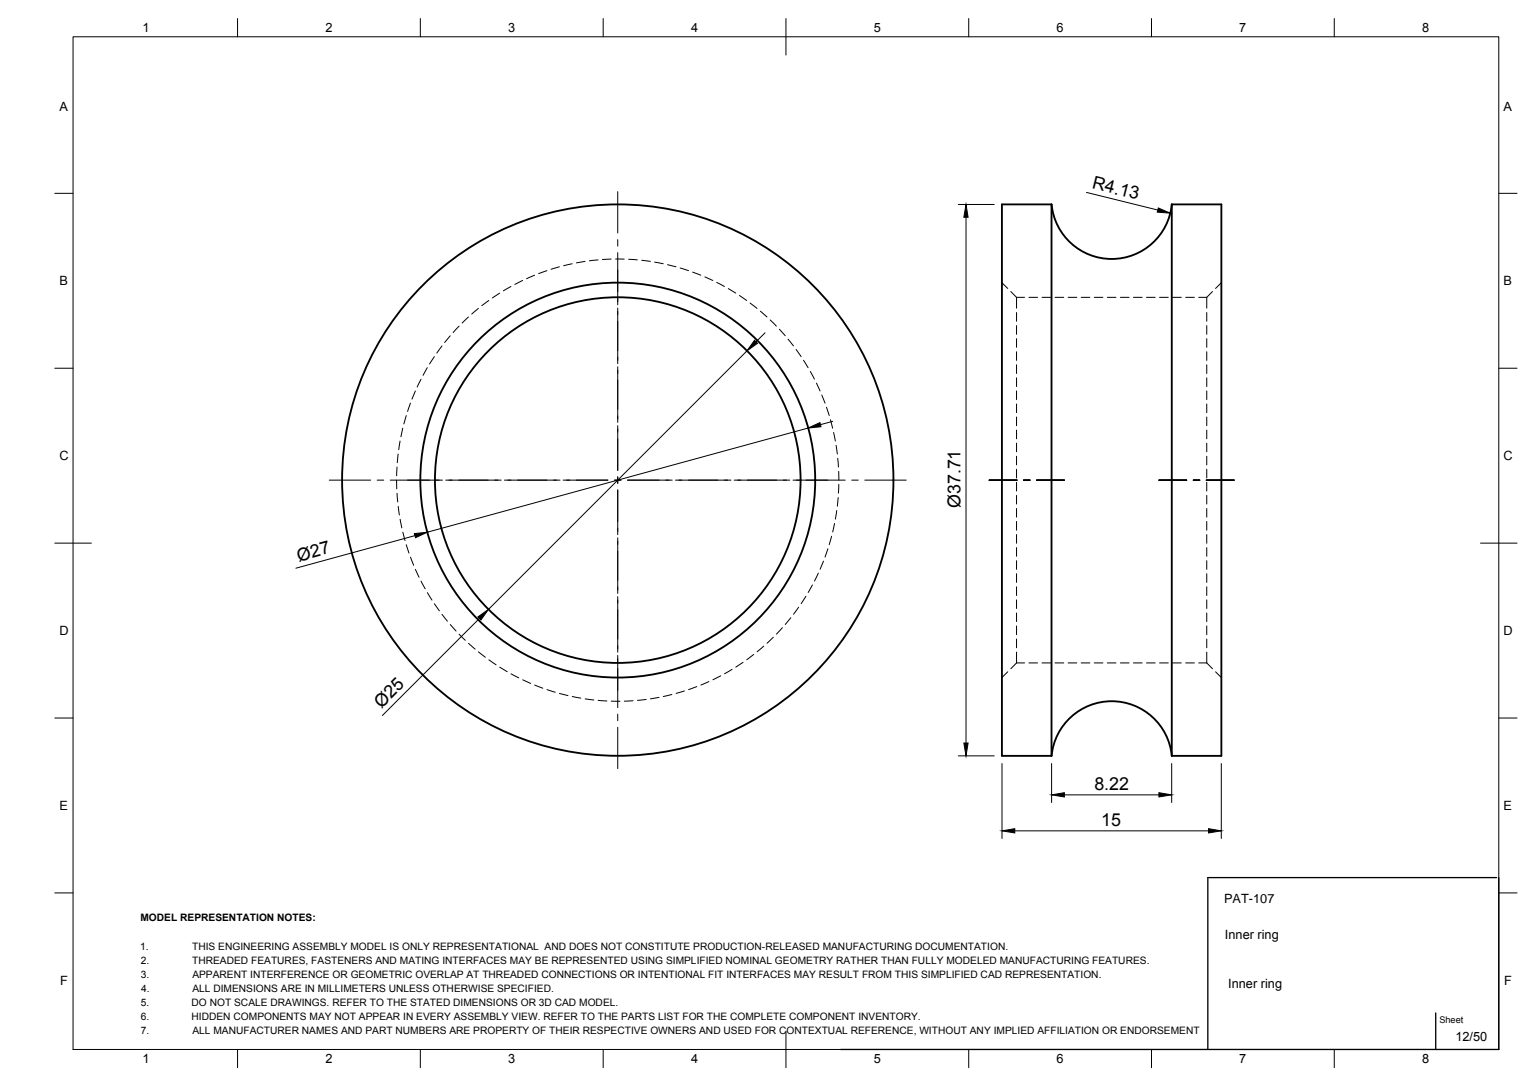
ISO-10303-21;
HEADER;
/* Generated by software containing ST-Developer
 * from STEP Tools, Inc. (www.steptools.com) 
 */

FILE_DESCRIPTION(
/* description */ ('Turntable on roller ring'),
/* implementation_level */ '2;1');

FILE_NAME(
/* name */ 'Inner ring.step',
/* time_stamp */ '2026-10-28T03:23:59-07:00',
/* author */ (''),
/* organization */ (''),
/* preprocessor_version */ 'ST-DEVELOPER v20.2',
/* originating_system */ 'Autodesk Translation Framework v15.17.0.0',
/* authorisation */ '');

FILE_SCHEMA (('AUTOMOTIVE_DESIGN { 1 0 10303 214 3 1 1 }'));
ENDSEC;

DATA;
#10=MECHANICAL_DESIGN_GEOMETRIC_PRESENTATION_REPRESENTATION('',(#621),#16281);
#472=TOROIDAL_SURFACE('',#9232,1.925,0.412776);
#479=CONICAL_SURFACE('',#9243,1.3,0.785398163397449);
#480=CONICAL_SURFACE('',#9250,1.3,0.785398163397449);
#511=SHAPE_REPRESENTATION_RELATIONSHIP('SRR','None',#16526,#566);
#566=ADVANCED_BREP_SHAPE_REPRESENTATION('',(#692),#16220);
#621=STYLED_ITEM('',(#16932),#692);
#692=MANIFOLD_SOLID_BREP('Body1',#8363);
#824=FACE_BOUND('',#1909,.T.);
#825=FACE_BOUND('',#1912,.T.);
#1021=PLANE('',#9245);
#1022=PLANE('',#9248);
#1332=FACE_OUTER_BOUND('',#1904,.T.);
#1333=FACE_OUTER_BOUND('',#1905,.T.);
#1334=FACE_OUTER_BOUND('',#1906,.T.);
#1335=FACE_OUTER_BOUND('',#1907,.T.);
#1336=FACE_OUTER_BOUND('',#1908,.T.);
#1337=FACE_OUTER_BOUND('',#1910,.T.);
#1338=FACE_OUTER_BOUND('',#1911,.T.);
#1339=FACE_OUTER_BOUND('',#1913,.T.);
#1904=EDGE_LOOP('',(#6019,#6020,#6021,#6022,#6023,#6024));
#1905=EDGE_LOOP('',(#6025,#6026,#6027,#6028,#6029));
#1906=EDGE_LOOP('',(#6030,#6031,#6032,#6033));
#1907=EDGE_LOOP('',(#6034,#6035,#6036,#6037));
#1908=EDGE_LOOP('',(#6038));
#1909=EDGE_LOOP('',(#6039));
#1910=EDGE_LOOP('',(#6040,#6041,#6042,#6043,#6044));
#1911=EDGE_LOOP('',(#6045));
#1912=EDGE_LOOP('',(#6046));
#1913=EDGE_LOOP('',(#6047,#6048,#6049,#6050));
#2578=LINE('',#13410,#3061);
#2579=LINE('',#13416,#3062);
#2580=LINE('',#13420,#3063);
#2581=LINE('',#13426,#3064);
#2582=LINE('',#13431,#3065);
#3061=VECTOR('',#10683,1.88531);
#3062=VECTOR('',#10690,1.25);
#3063=VECTOR('',#10695,1.3);
#3064=VECTOR('',#10704,1.88531);
#3065=VECTOR('',#10711,1.3);
#3561=CIRCLE('',#9233,1.88531);
#3562=CIRCLE('',#9234,1.88531);
#3563=CIRCLE('',#9235,0.412776);
#3564=CIRCLE('',#9236,1.88531);
#3565=CIRCLE('',#9237,1.88531);
#3566=CIRCLE('',#9239,1.88531);
#3567=CIRCLE('',#9241,1.25);
#3568=CIRCLE('',#9242,1.25);
#3569=CIRCLE('',#9244,1.35);
#3570=CIRCLE('',#9247,1.88531);
#3571=CIRCLE('',#9249,1.35);
#4067=VERTEX_POINT('',#13399);
#4068=VERTEX_POINT('',#13400);
#4069=VERTEX_POINT('',#13403);
#4070=VERTEX_POINT('',#13405);
#4071=VERTEX_POINT('',#13409);
#4072=VERTEX_POINT('',#13413);
#4073=VERTEX_POINT('',#13415);
#4074=VERTEX_POINT('',#13419);
#4075=VERTEX_POINT('',#13424);
#4076=VERTEX_POINT('',#13428);
#4820=EDGE_CURVE('',#4067,#4068,#3561,.T.);
#4821=EDGE_CURVE('',#4068,#4067,#3562,.T.);
#4822=EDGE_CURVE('',#4068,#4069,#3563,.T.);
#4823=EDGE_CURVE('',#4070,#4069,#3564,.T.);
#4824=EDGE_CURVE('',#4069,#4070,#3565,.T.);
#4825=EDGE_CURVE('',#4070,#4071,#2578,.T.);
#4826=EDGE_CURVE('',#4071,#4071,#3566,.T.);
#4827=EDGE_CURVE('',#4072,#4072,#3567,.T.);
#4828=EDGE_CURVE('',#4072,#4073,#2579,.T.);
#4829=EDGE_CURVE('',#4073,#4073,#3568,.T.);
#4830=EDGE_CURVE('',#4073,#4074,#2580,.T.);
#4831=EDGE_CURVE('',#4074,#4074,#3569,.T.);
#4832=EDGE_CURVE('',#4075,#4075,#3570,.T.);
#4833=EDGE_CURVE('',#4075,#4067,#2581,.T.);
#4834=EDGE_CURVE('',#4076,#4076,#3571,.T.);
#4835=EDGE_CURVE('',#4076,#4072,#2582,.T.);
#6019=ORIENTED_EDGE('',*,*,#4820,.F.);
#6020=ORIENTED_EDGE('',*,*,#4821,.F.);
#6021=ORIENTED_EDGE('',*,*,#4822,.T.);
#6022=ORIENTED_EDGE('',*,*,#4823,.F.);
#6023=ORIENTED_EDGE('',*,*,#4824,.F.);
#6024=ORIENTED_EDGE('',*,*,#4822,.F.);
#6025=ORIENTED_EDGE('',*,*,#4823,.T.);
#6026=ORIENTED_EDGE('',*,*,#4824,.T.);
#6027=ORIENTED_EDGE('',*,*,#4825,.T.);
#6028=ORIENTED_EDGE('',*,*,#4826,.T.);
#6029=ORIENTED_EDGE('',*,*,#4825,.F.);
#6030=ORIENTED_EDGE('',*,*,#4827,.T.);
#6031=ORIENTED_EDGE('',*,*,#4828,.T.);
#6032=ORIENTED_EDGE('',*,*,#4829,.F.);
#6033=ORIENTED_EDGE('',*,*,#4828,.F.);
#6034=ORIENTED_EDGE('',*,*,#4829,.T.);
#6035=ORIENTED_EDGE('',*,*,#4830,.T.);
#6036=ORIENTED_EDGE('',*,*,#4831,.F.);
#6037=ORIENTED_EDGE('',*,*,#4830,.F.);
#6038=ORIENTED_EDGE('',*,*,#4826,.F.);
#6039=ORIENTED_EDGE('',*,*,#4831,.T.);
#6040=ORIENTED_EDGE('',*,*,#4832,.F.);
#6041=ORIENTED_EDGE('',*,*,#4833,.T.);
#6042=ORIENTED_EDGE('',*,*,#4820,.T.);
#6043=ORIENTED_EDGE('',*,*,#4821,.T.);
#6044=ORIENTED_EDGE('',*,*,#4833,.F.);
#6045=ORIENTED_EDGE('',*,*,#4832,.T.);
#6046=ORIENTED_EDGE('',*,*,#4834,.F.);
#6047=ORIENTED_EDGE('',*,*,#4834,.T.);
#6048=ORIENTED_EDGE('',*,*,#4835,.T.);
#6049=ORIENTED_EDGE('',*,*,#4827,.F.);
#6050=ORIENTED_EDGE('',*,*,#4835,.F.);
#7717=CYLINDRICAL_SURFACE('',#9238,1.88531);
#7718=CYLINDRICAL_SURFACE('',#9240,1.25);
#7719=CYLINDRICAL_SURFACE('',#9246,1.88531);
#7935=ADVANCED_FACE('',(#1332),#472,.F.);
#7936=ADVANCED_FACE('',(#1333),#7717,.T.);
#7937=ADVANCED_FACE('',(#1334),#7718,.F.);
#7938=ADVANCED_FACE('',(#1335),#479,.F.);
#7939=ADVANCED_FACE('',(#1336,#824),#1021,.T.);
#7940=ADVANCED_FACE('',(#1337),#7719,.T.);
#7941=ADVANCED_FACE('',(#1338,#825),#1022,.T.);
#7942=ADVANCED_FACE('',(#1339),#480,.F.);
#8363=CLOSED_SHELL('',(#7935,#7936,#7937,#7938,#7939,#7940,#7941,#7942));
#9231=AXIS2_PLACEMENT_3D('',#13397,#10667,#10668);
#9232=AXIS2_PLACEMENT_3D('',#13398,#10669,#10670);
#9233=AXIS2_PLACEMENT_3D('',#13401,#10671,#10672);
#9234=AXIS2_PLACEMENT_3D('',#13402,#10673,#10674);
#9235=AXIS2_PLACEMENT_3D('',#13404,#10675,#10676);
#9236=AXIS2_PLACEMENT_3D('',#13406,#10677,#10678);
#9237=AXIS2_PLACEMENT_3D('',#13407,#10679,#10680);
#9238=AXIS2_PLACEMENT_3D('',#13408,#10681,#10682);
#9239=AXIS2_PLACEMENT_3D('',#13411,#10684,#10685);
#9240=AXIS2_PLACEMENT_3D('',#13412,#10686,#10687);
#9241=AXIS2_PLACEMENT_3D('',#13414,#10688,#10689);
#9242=AXIS2_PLACEMENT_3D('',#13417,#10691,#10692);
#9243=AXIS2_PLACEMENT_3D('',#13418,#10693,#10694);
#9244=AXIS2_PLACEMENT_3D('',#13421,#10696,#10697);
#9245=AXIS2_PLACEMENT_3D('',#13422,#10698,#10699);
#9246=AXIS2_PLACEMENT_3D('',#13423,#10700,#10701);
#9247=AXIS2_PLACEMENT_3D('',#13425,#10702,#10703);
#9248=AXIS2_PLACEMENT_3D('',#13427,#10705,#10706);
#9249=AXIS2_PLACEMENT_3D('',#13429,#10707,#10708);
#9250=AXIS2_PLACEMENT_3D('',#13430,#10709,#10710);
#10667=DIRECTION('axis',(0.,0.,1.));
#10668=DIRECTION('refdir',(1.,0.,0.));
#10669=DIRECTION('center_axis',(0.,-1.,0.));
#10670=DIRECTION('ref_axis',(0.,0.,-1.));
#10671=DIRECTION('center_axis',(0.,-1.,0.));
#10672=DIRECTION('ref_axis',(1.,0.,0.));
#10673=DIRECTION('center_axis',(0.,-1.,0.));
#10674=DIRECTION('ref_axis',(1.,0.,0.));
#10675=DIRECTION('center_axis',(1.,0.,1.22464679914735E-16));
#10676=DIRECTION('ref_axis',(-1.22464679914735E-16,0.,1.));
#10677=DIRECTION('center_axis',(0.,1.,0.));
#10678=DIRECTION('ref_axis',(1.,0.,0.));
#10679=DIRECTION('center_axis',(0.,1.,0.));
#10680=DIRECTION('ref_axis',(1.,0.,0.));
#10681=DIRECTION('center_axis',(0.,-1.,0.));
#10682=DIRECTION('ref_axis',(1.,0.,0.));
#10683=DIRECTION('',(0.,1.,0.));
#10684=DIRECTION('center_axis',(0.,-1.,0.));
#10685=DIRECTION('ref_axis',(1.,0.,0.));
#10686=DIRECTION('center_axis',(0.,-1.,0.));
#10687=DIRECTION('ref_axis',(1.,0.,0.));
#10688=DIRECTION('center_axis',(0.,-1.,0.));
#10689=DIRECTION('ref_axis',(1.,0.,0.));
#10690=DIRECTION('',(0.,1.,0.));
#10691=DIRECTION('center_axis',(0.,-1.,0.));
#10692=DIRECTION('ref_axis',(1.,0.,0.));
#10693=DIRECTION('center_axis',(0.,1.,0.));
#10694=DIRECTION('ref_axis',(1.,0.,0.));
#10695=DIRECTION('',(-0.707106781186548,0.707106781186547,-8.65956056235494E-17));
#10696=DIRECTION('center_axis',(0.,-1.,0.));
#10697=DIRECTION('ref_axis',(1.,0.,0.));
#10698=DIRECTION('center_axis',(0.,1.,0.));
#10699=DIRECTION('ref_axis',(0.,0.,1.));
#10700=DIRECTION('center_axis',(0.,-1.,0.));
#10701=DIRECTION('ref_axis',(1.,0.,0.));
#10702=DIRECTION('center_axis',(0.,-1.,0.));
#10703=DIRECTION('ref_axis',(1.,0.,0.));
#10704=DIRECTION('',(0.,1.,0.));
#10705=DIRECTION('center_axis',(0.,-1.,0.));
#10706=DIRECTION('ref_axis',(0.,0.,-1.));
#10707=DIRECTION('center_axis',(0.,-1.,0.));
#10708=DIRECTION('ref_axis',(1.,0.,0.));
#10709=DIRECTION('center_axis',(0.,-1.,0.));
#10710=DIRECTION('ref_axis',(1.,0.,0.));
#10711=DIRECTION('',(0.707106781186548,0.707106781186547,8.65956056235494E-17));
#13397=CARTESIAN_POINT('',(0.,0.,0.));
#13398=CARTESIAN_POINT('Origin',(0.,0.,0.));
#13399=CARTESIAN_POINT('',(-1.88531,-0.410863395882378,-2.3088388569005E-16));
#13400=CARTESIAN_POINT('',(-2.3088388569005E-16,-0.410863395882378,1.88531));
#13401=CARTESIAN_POINT('Origin',(0.,-0.410863395882378,0.));
#13402=CARTESIAN_POINT('Origin',(0.,-0.410863395882378,0.));
#13403=CARTESIAN_POINT('',(-2.3088388569005E-16,0.410863395882378,1.88531));
#13404=CARTESIAN_POINT('Origin',(-2.35744508835865E-16,0.,1.925));
#13405=CARTESIAN_POINT('',(-1.88531,0.410863395882378,2.3088388569005E-16));
#13406=CARTESIAN_POINT('Origin',(0.,0.410863395882378,0.));
#13407=CARTESIAN_POINT('Origin',(0.,0.410863395882378,0.));
#13408=CARTESIAN_POINT('Origin',(0.,0.,0.));
#13409=CARTESIAN_POINT('',(-1.88531,0.75,-2.3088388569005E-16));
#13410=CARTESIAN_POINT('',(-1.88531,0.,-2.3088388569005E-16));
#13411=CARTESIAN_POINT('Origin',(0.,0.75,0.));
#13412=CARTESIAN_POINT('Origin',(0.,0.,0.));
#13413=CARTESIAN_POINT('',(-1.25,-0.65,-1.53080849893419E-16));
#13414=CARTESIAN_POINT('Origin',(0.,-0.65,0.));
#13415=CARTESIAN_POINT('',(-1.25,0.65,-1.53080849893419E-16));
#13416=CARTESIAN_POINT('',(-1.25,0.,-1.53080849893419E-16));
#13417=CARTESIAN_POINT('Origin',(0.,0.65,0.));
#13418=CARTESIAN_POINT('Origin',(0.,0.7,0.));
#13419=CARTESIAN_POINT('',(-1.35,0.75,-1.65327317884893E-16));
#13420=CARTESIAN_POINT('',(-1.3,0.7,-1.59204083889156E-16));
#13421=CARTESIAN_POINT('Origin',(0.,0.75,0.));
#13422=CARTESIAN_POINT('Origin',(1.88531,0.75,0.));
#13423=CARTESIAN_POINT('Origin',(0.,0.,0.));
#13424=CARTESIAN_POINT('',(-1.88531,-0.75,-2.3088388569005E-16));
#13425=CARTESIAN_POINT('Origin',(0.,-0.75,0.));
#13426=CARTESIAN_POINT('',(-1.88531,0.,-2.3088388569005E-16));
#13427=CARTESIAN_POINT('Origin',(1.35,-0.75,0.));
#13428=CARTESIAN_POINT('',(-1.35,-0.75,-1.65327317884893E-16));
#13429=CARTESIAN_POINT('Origin',(0.,-0.75,0.));
#13430=CARTESIAN_POINT('Origin',(0.,-0.7,0.));
#13431=CARTESIAN_POINT('',(-1.3,-0.7,-1.59204083889156E-16));
#16151=UNCERTAINTY_MEASURE_WITH_UNIT(LENGTH_MEASURE(0.001),#16282,
'DISTANCE_ACCURACY_VALUE',
'Maximum model space distance between geometric entities at asserted c
onnectivities');
#16212=UNCERTAINTY_MEASURE_WITH_UNIT(LENGTH_MEASURE(0.001),#16282,
'DISTANCE_ACCURACY_VALUE',
'Maximum model space distance between geometric entities at asserted c
onnectivities');
#16220=(
GEOMETRIC_REPRESENTATION_CONTEXT(3)
GLOBAL_UNCERTAINTY_ASSIGNED_CONTEXT((#16151))
GLOBAL_UNIT_ASSIGNED_CONTEXT((#16282,#16284,#16285))
REPRESENTATION_CONTEXT('','3D')
);
#16281=(
GEOMETRIC_REPRESENTATION_CONTEXT(3)
GLOBAL_UNCERTAINTY_ASSIGNED_CONTEXT((#16212))
GLOBAL_UNIT_ASSIGNED_CONTEXT((#16282,#16284,#16285))
REPRESENTATION_CONTEXT('','3D')
);
#16282=(
LENGTH_UNIT()
NAMED_UNIT(*)
SI_UNIT(.CENTI.,.METRE.)
);
#16284=(
NAMED_UNIT(*)
PLANE_ANGLE_UNIT()
SI_UNIT($,.RADIAN.)
);
#16285=(
NAMED_UNIT(*)
SI_UNIT($,.STERADIAN.)
SOLID_ANGLE_UNIT()
);
#16293=SHAPE_DEFINITION_REPRESENTATION(#16361,#16526);
#16361=PRODUCT_DEFINITION_SHAPE('',$,#16595);
#16526=SHAPE_REPRESENTATION('',(#9231),#16220);
#16587=PRODUCT_DEFINITION_CONTEXT('part definition',#16793,'design');
#16595=PRODUCT_DEFINITION('Inner ring','Inner ring',#16663,#16587);
#16663=PRODUCT_DEFINITION_FORMATION('',$,#16802);
#16793=APPLICATION_CONTEXT(
'Core Data for Automotive Mechanical Design Process');
#16794=PRODUCT_CONTEXT('part definition',#16793,'mechanical');
#16802=PRODUCT('Inner ring','Inner ring','Inner ring',(#16794));
#16926=COLOUR_RGB('Grey',0.48,0.52,0.57);
#16927=FILL_AREA_STYLE_COLOUR('',#16926);
#16928=FILL_AREA_STYLE('',(#16927));
#16929=SURFACE_STYLE_FILL_AREA(#16928);
#16930=SURFACE_SIDE_STYLE('',(#16929));
#16931=SURFACE_STYLE_USAGE(.BOTH.,#16930);
#16932=PRESENTATION_STYLE_ASSIGNMENT((#16931));
ENDSEC;
END-ISO-10303-21;
